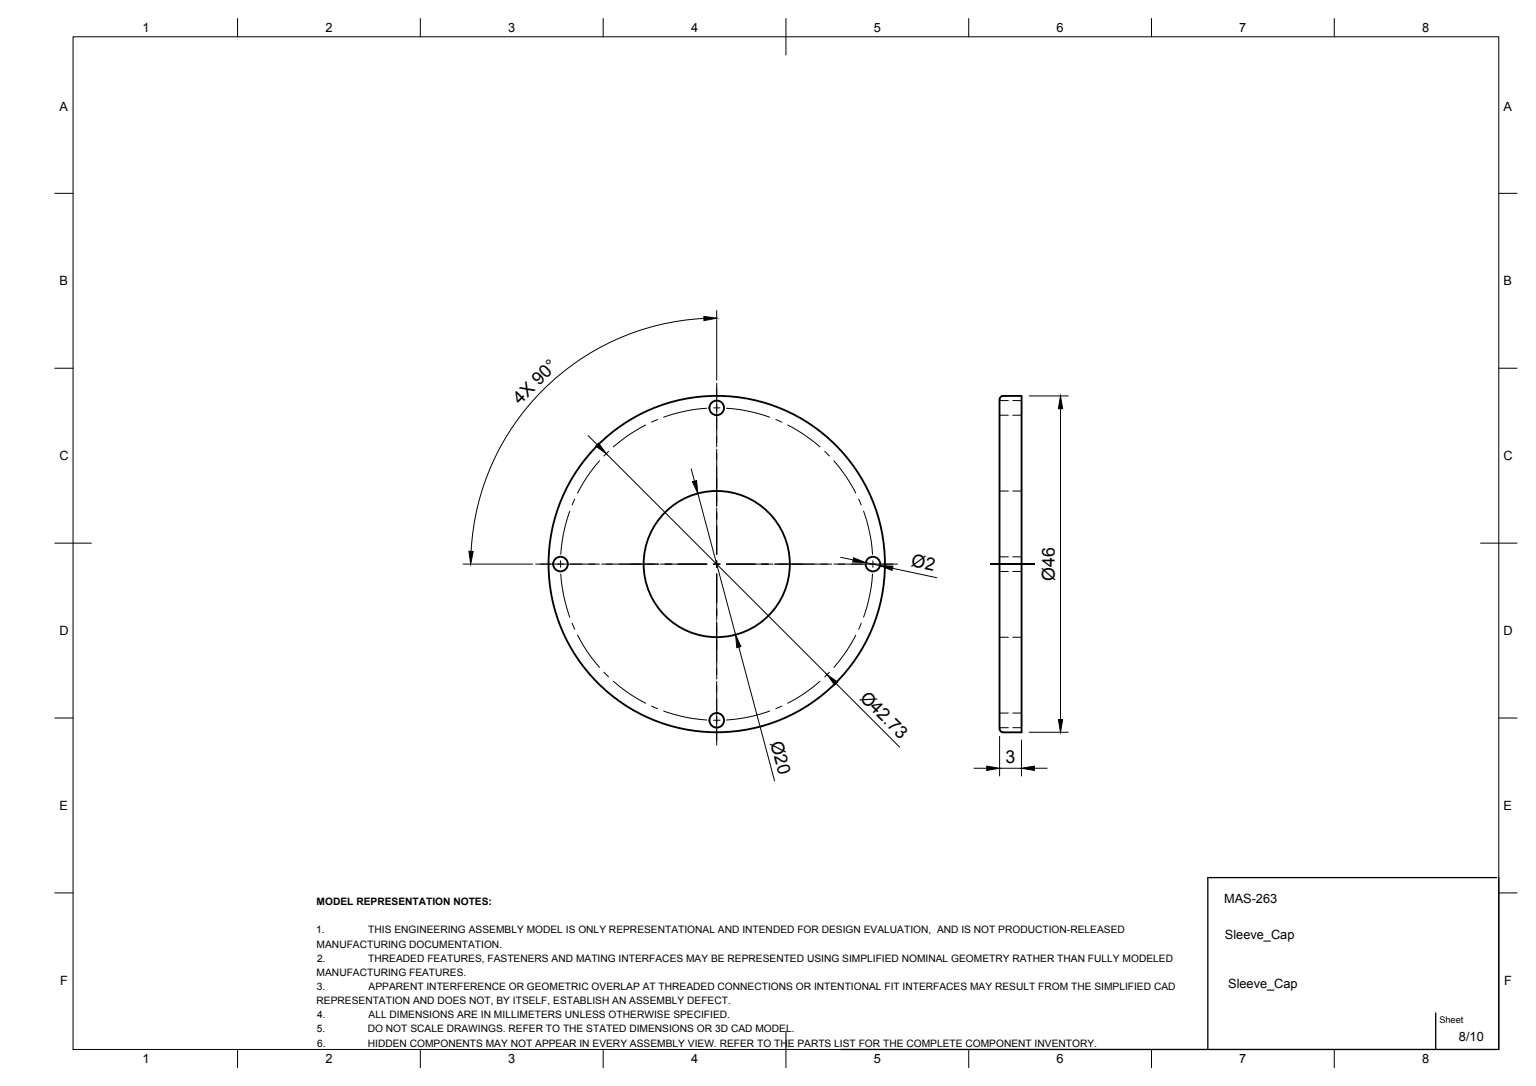
ISO-10303-21;
HEADER;
/* Generated by software containing ST-Developer
 * from STEP Tools, Inc. (www.steptools.com) 
 */

FILE_DESCRIPTION(
/* description */ (''),
/* implementation_level */ '2;1');

FILE_NAME(
/* name */ 'Sleeve_Cap.step',
/* time_stamp */ '2026-10-12T15:47:30-07:00',
/* author */ (''),
/* organization */ (''),
/* preprocessor_version */ 'ST-DEVELOPER v20.2',
/* originating_system */ 'Autodesk Translation Framework v15.15.0.0',
/* authorisation */ '');

FILE_SCHEMA (('AUTOMOTIVE_DESIGN { 1 0 10303 214 3 1 1 }'));
ENDSEC;

DATA;
#10=MECHANICAL_DESIGN_GEOMETRIC_PRESENTATION_REPRESENTATION('',(#86),#88483);
#68=SHAPE_REPRESENTATION_RELATIONSHIP('SRR','None',#88524,#77);
#77=ADVANCED_BREP_SHAPE_REPRESENTATION('',(#121),#88478);
#86=STYLED_ITEM('',(#88574),#121);
#121=MANIFOLD_SOLID_BREP('Body1',#12996);
#173=TOROIDAL_SURFACE('',#13852,22.5,0.5);
#368=FACE_BOUND('',#1937,.T.);
#369=FACE_BOUND('',#1938,.T.);
#370=FACE_BOUND('',#1939,.T.);
#371=FACE_BOUND('',#1940,.T.);
#372=FACE_BOUND('',#1941,.T.);
#373=FACE_BOUND('',#1948,.T.);
#374=FACE_BOUND('',#1949,.T.);
#375=FACE_BOUND('',#1950,.T.);
#376=FACE_BOUND('',#1951,.T.);
#377=FACE_BOUND('',#1952,.T.);
#523=PLANE('',#13859);
#524=PLANE('',#13875);
#1247=FACE_OUTER_BOUND('',#1934,.T.);
#1248=FACE_OUTER_BOUND('',#1935,.T.);
#1249=FACE_OUTER_BOUND('',#1936,.T.);
#1250=FACE_OUTER_BOUND('',#1942,.T.);
#1251=FACE_OUTER_BOUND('',#1943,.T.);
#1252=FACE_OUTER_BOUND('',#1944,.T.);
#1253=FACE_OUTER_BOUND('',#1945,.T.);
#1254=FACE_OUTER_BOUND('',#1946,.T.);
#1255=FACE_OUTER_BOUND('',#1947,.T.);
#1934=EDGE_LOOP('',(#11196,#11197,#11198,#11199,#11200));
#1935=EDGE_LOOP('',(#11201,#11202,#11203,#11204,#11205));
#1936=EDGE_LOOP('',(#11206));
#1937=EDGE_LOOP('',(#11207));
#1938=EDGE_LOOP('',(#11208));
#1939=EDGE_LOOP('',(#11209));
#1940=EDGE_LOOP('',(#11210));
#1941=EDGE_LOOP('',(#11211));
#1942=EDGE_LOOP('',(#11212,#11213,#11214,#11215));
#1943=EDGE_LOOP('',(#11216,#11217,#11218,#11219));
#1944=EDGE_LOOP('',(#11220,#11221,#11222,#11223));
#1945=EDGE_LOOP('',(#11224,#11225,#11226,#11227));
#1946=EDGE_LOOP('',(#11228,#11229,#11230,#11231));
#1947=EDGE_LOOP('',(#11232));
#1948=EDGE_LOOP('',(#11233));
#1949=EDGE_LOOP('',(#11234));
#1950=EDGE_LOOP('',(#11235));
#1951=EDGE_LOOP('',(#11236));
#1952=EDGE_LOOP('',(#11237));
#2625=CIRCLE('',#13853,22.5);
#2626=CIRCLE('',#13854,0.5);
#2627=CIRCLE('',#13855,23.);
#2628=CIRCLE('',#13856,23.);
#2629=CIRCLE('',#13858,23.);
#2630=CIRCLE('',#13860,1.);
#2631=CIRCLE('',#13861,1.);
#2632=CIRCLE('',#13862,1.);
#2633=CIRCLE('',#13863,1.);
#2634=CIRCLE('',#13864,10.);
#2635=CIRCLE('',#13866,1.);
#2636=CIRCLE('',#13868,1.);
#2637=CIRCLE('',#13870,1.);
#2638=CIRCLE('',#13872,1.);
#2639=CIRCLE('',#13874,10.);
#4028=LINE('',#87095,#4498);
#4029=LINE('',#87110,#4499);
#4030=LINE('',#87114,#4500);
#4031=LINE('',#87118,#4501);
#4032=LINE('',#87122,#4502);
#4033=LINE('',#87127,#4503);
#4498=VECTOR('',#16194,23.);
#4499=VECTOR('',#16211,1.);
#4500=VECTOR('',#16216,1.);
#4501=VECTOR('',#16221,1.);
#4502=VECTOR('',#16226,1.);
#4503=VECTOR('',#16233,10.);
#5737=VERTEX_POINT('',#87086);
#5738=VERTEX_POINT('',#87088);
#5739=VERTEX_POINT('',#87090);
#5740=VERTEX_POINT('',#87094);
#5741=VERTEX_POINT('',#87098);
#5742=VERTEX_POINT('',#87100);
#5743=VERTEX_POINT('',#87102);
#5744=VERTEX_POINT('',#87104);
#5745=VERTEX_POINT('',#87106);
#5746=VERTEX_POINT('',#87109);
#5747=VERTEX_POINT('',#87113);
#5748=VERTEX_POINT('',#87117);
#5749=VERTEX_POINT('',#87121);
#5750=VERTEX_POINT('',#87125);
#7610=EDGE_CURVE('',#5737,#5737,#2625,.T.);
#7611=EDGE_CURVE('',#5737,#5738,#2626,.T.);
#7612=EDGE_CURVE('',#5738,#5739,#2627,.T.);
#7613=EDGE_CURVE('',#5739,#5738,#2628,.T.);
#7614=EDGE_CURVE('',#5739,#5740,#4028,.T.);
#7615=EDGE_CURVE('',#5740,#5740,#2629,.T.);
#7616=EDGE_CURVE('',#5741,#5741,#2630,.T.);
#7617=EDGE_CURVE('',#5742,#5742,#2631,.T.);
#7618=EDGE_CURVE('',#5743,#5743,#2632,.T.);
#7619=EDGE_CURVE('',#5744,#5744,#2633,.T.);
#7620=EDGE_CURVE('',#5745,#5745,#2634,.T.);
#7621=EDGE_CURVE('',#5741,#5746,#4029,.T.);
#7622=EDGE_CURVE('',#5746,#5746,#2635,.T.);
#7623=EDGE_CURVE('',#5742,#5747,#4030,.T.);
#7624=EDGE_CURVE('',#5747,#5747,#2636,.T.);
#7625=EDGE_CURVE('',#5743,#5748,#4031,.T.);
#7626=EDGE_CURVE('',#5748,#5748,#2637,.T.);
#7627=EDGE_CURVE('',#5744,#5749,#4032,.T.);
#7628=EDGE_CURVE('',#5749,#5749,#2638,.T.);
#7629=EDGE_CURVE('',#5750,#5750,#2639,.T.);
#7630=EDGE_CURVE('',#5750,#5745,#4033,.T.);
#11196=ORIENTED_EDGE('',*,*,#7610,.T.);
#11197=ORIENTED_EDGE('',*,*,#7611,.T.);
#11198=ORIENTED_EDGE('',*,*,#7612,.T.);
#11199=ORIENTED_EDGE('',*,*,#7613,.T.);
#11200=ORIENTED_EDGE('',*,*,#7611,.F.);
#11201=ORIENTED_EDGE('',*,*,#7613,.F.);
#11202=ORIENTED_EDGE('',*,*,#7614,.T.);
#11203=ORIENTED_EDGE('',*,*,#7615,.T.);
#11204=ORIENTED_EDGE('',*,*,#7614,.F.);
#11205=ORIENTED_EDGE('',*,*,#7612,.F.);
#11206=ORIENTED_EDGE('',*,*,#7610,.F.);
#11207=ORIENTED_EDGE('',*,*,#7616,.T.);
#11208=ORIENTED_EDGE('',*,*,#7617,.T.);
#11209=ORIENTED_EDGE('',*,*,#7618,.T.);
#11210=ORIENTED_EDGE('',*,*,#7619,.T.);
#11211=ORIENTED_EDGE('',*,*,#7620,.T.);
#11212=ORIENTED_EDGE('',*,*,#7616,.F.);
#11213=ORIENTED_EDGE('',*,*,#7621,.T.);
#11214=ORIENTED_EDGE('',*,*,#7622,.F.);
#11215=ORIENTED_EDGE('',*,*,#7621,.F.);
#11216=ORIENTED_EDGE('',*,*,#7617,.F.);
#11217=ORIENTED_EDGE('',*,*,#7623,.T.);
#11218=ORIENTED_EDGE('',*,*,#7624,.F.);
#11219=ORIENTED_EDGE('',*,*,#7623,.F.);
#11220=ORIENTED_EDGE('',*,*,#7618,.F.);
#11221=ORIENTED_EDGE('',*,*,#7625,.T.);
#11222=ORIENTED_EDGE('',*,*,#7626,.F.);
#11223=ORIENTED_EDGE('',*,*,#7625,.F.);
#11224=ORIENTED_EDGE('',*,*,#7619,.F.);
#11225=ORIENTED_EDGE('',*,*,#7627,.T.);
#11226=ORIENTED_EDGE('',*,*,#7628,.F.);
#11227=ORIENTED_EDGE('',*,*,#7627,.F.);
#11228=ORIENTED_EDGE('',*,*,#7629,.T.);
#11229=ORIENTED_EDGE('',*,*,#7630,.T.);
#11230=ORIENTED_EDGE('',*,*,#7620,.F.);
#11231=ORIENTED_EDGE('',*,*,#7630,.F.);
#11232=ORIENTED_EDGE('',*,*,#7615,.F.);
#11233=ORIENTED_EDGE('',*,*,#7629,.F.);
#11234=ORIENTED_EDGE('',*,*,#7628,.T.);
#11235=ORIENTED_EDGE('',*,*,#7626,.T.);
#11236=ORIENTED_EDGE('',*,*,#7624,.T.);
#11237=ORIENTED_EDGE('',*,*,#7622,.T.);
#12245=CYLINDRICAL_SURFACE('',#13857,23.);
#12246=CYLINDRICAL_SURFACE('',#13865,1.);
#12247=CYLINDRICAL_SURFACE('',#13867,1.);
#12248=CYLINDRICAL_SURFACE('',#13869,1.);
#12249=CYLINDRICAL_SURFACE('',#13871,1.);
#12250=CYLINDRICAL_SURFACE('',#13873,10.);
#12777=ADVANCED_FACE('',(#1247),#173,.T.);
#12778=ADVANCED_FACE('',(#1248),#12245,.T.);
#12779=ADVANCED_FACE('',(#1249,#368,#369,#370,#371,#372),#523,.T.);
#12780=ADVANCED_FACE('',(#1250),#12246,.F.);
#12781=ADVANCED_FACE('',(#1251),#12247,.F.);
#12782=ADVANCED_FACE('',(#1252),#12248,.F.);
#12783=ADVANCED_FACE('',(#1253),#12249,.F.);
#12784=ADVANCED_FACE('',(#1254),#12250,.F.);
#12785=ADVANCED_FACE('',(#1255,#373,#374,#375,#376,#377),#524,.F.);
#12996=CLOSED_SHELL('',(#12777,#12778,#12779,#12780,#12781,#12782,#12783,
#12784,#12785));
#13851=AXIS2_PLACEMENT_3D('',#87084,#16180,#16181);
#13852=AXIS2_PLACEMENT_3D('',#87085,#16182,#16183);
#13853=AXIS2_PLACEMENT_3D('',#87087,#16184,#16185);
#13854=AXIS2_PLACEMENT_3D('',#87089,#16186,#16187);
#13855=AXIS2_PLACEMENT_3D('',#87091,#16188,#16189);
#13856=AXIS2_PLACEMENT_3D('',#87092,#16190,#16191);
#13857=AXIS2_PLACEMENT_3D('',#87093,#16192,#16193);
#13858=AXIS2_PLACEMENT_3D('',#87096,#16195,#16196);
#13859=AXIS2_PLACEMENT_3D('',#87097,#16197,#16198);
#13860=AXIS2_PLACEMENT_3D('',#87099,#16199,#16200);
#13861=AXIS2_PLACEMENT_3D('',#87101,#16201,#16202);
#13862=AXIS2_PLACEMENT_3D('',#87103,#16203,#16204);
#13863=AXIS2_PLACEMENT_3D('',#87105,#16205,#16206);
#13864=AXIS2_PLACEMENT_3D('',#87107,#16207,#16208);
#13865=AXIS2_PLACEMENT_3D('',#87108,#16209,#16210);
#13866=AXIS2_PLACEMENT_3D('',#87111,#16212,#16213);
#13867=AXIS2_PLACEMENT_3D('',#87112,#16214,#16215);
#13868=AXIS2_PLACEMENT_3D('',#87115,#16217,#16218);
#13869=AXIS2_PLACEMENT_3D('',#87116,#16219,#16220);
#13870=AXIS2_PLACEMENT_3D('',#87119,#16222,#16223);
#13871=AXIS2_PLACEMENT_3D('',#87120,#16224,#16225);
#13872=AXIS2_PLACEMENT_3D('',#87123,#16227,#16228);
#13873=AXIS2_PLACEMENT_3D('',#87124,#16229,#16230);
#13874=AXIS2_PLACEMENT_3D('',#87126,#16231,#16232);
#13875=AXIS2_PLACEMENT_3D('',#87128,#16234,#16235);
#16180=DIRECTION('axis',(0.,0.,1.));
#16181=DIRECTION('refdir',(1.,0.,0.));
#16182=DIRECTION('center_axis',(0.,0.,1.));
#16183=DIRECTION('ref_axis',(1.,0.,0.));
#16184=DIRECTION('center_axis',(0.,0.,-1.));
#16185=DIRECTION('ref_axis',(-1.,0.,0.));
#16186=DIRECTION('center_axis',(1.22464679914735E-16,-1.,0.));
#16187=DIRECTION('ref_axis',(-1.,-1.22464679914735E-16,0.));
#16188=DIRECTION('center_axis',(0.,0.,1.));
#16189=DIRECTION('ref_axis',(-1.,0.,0.));
#16190=DIRECTION('center_axis',(0.,0.,1.));
#16191=DIRECTION('ref_axis',(-1.,0.,0.));
#16192=DIRECTION('center_axis',(0.,0.,1.));
#16193=DIRECTION('ref_axis',(-1.,0.,0.));
#16194=DIRECTION('',(0.,0.,-1.));
#16195=DIRECTION('center_axis',(0.,0.,1.));
#16196=DIRECTION('ref_axis',(-1.,0.,0.));
#16197=DIRECTION('center_axis',(0.,0.,1.));
#16198=DIRECTION('ref_axis',(-1.,0.,0.));
#16199=DIRECTION('center_axis',(0.,0.,-1.));
#16200=DIRECTION('ref_axis',(-1.,0.,0.));
#16201=DIRECTION('center_axis',(0.,0.,-1.));
#16202=DIRECTION('ref_axis',(-1.,0.,0.));
#16203=DIRECTION('center_axis',(0.,0.,-1.));
#16204=DIRECTION('ref_axis',(-1.,0.,0.));
#16205=DIRECTION('center_axis',(0.,0.,-1.));
#16206=DIRECTION('ref_axis',(-1.,0.,0.));
#16207=DIRECTION('center_axis',(0.,0.,-1.));
#16208=DIRECTION('ref_axis',(-1.,0.,0.));
#16209=DIRECTION('center_axis',(0.,0.,-1.));
#16210=DIRECTION('ref_axis',(-1.,0.,0.));
#16211=DIRECTION('',(0.,0.,-1.));
#16212=DIRECTION('center_axis',(0.,0.,1.));
#16213=DIRECTION('ref_axis',(-1.,0.,0.));
#16214=DIRECTION('center_axis',(0.,0.,-1.));
#16215=DIRECTION('ref_axis',(-1.,0.,0.));
#16216=DIRECTION('',(0.,0.,-1.));
#16217=DIRECTION('center_axis',(0.,0.,1.));
#16218=DIRECTION('ref_axis',(-1.,0.,0.));
#16219=DIRECTION('center_axis',(0.,0.,-1.));
#16220=DIRECTION('ref_axis',(-1.,0.,0.));
#16221=DIRECTION('',(0.,0.,-1.));
#16222=DIRECTION('center_axis',(0.,0.,1.));
#16223=DIRECTION('ref_axis',(-1.,0.,0.));
#16224=DIRECTION('center_axis',(0.,0.,-1.));
#16225=DIRECTION('ref_axis',(-1.,0.,0.));
#16226=DIRECTION('',(0.,0.,-1.));
#16227=DIRECTION('center_axis',(0.,0.,1.));
#16228=DIRECTION('ref_axis',(-1.,0.,0.));
#16229=DIRECTION('center_axis',(0.,0.,1.));
#16230=DIRECTION('ref_axis',(-1.,0.,0.));
#16231=DIRECTION('center_axis',(0.,0.,-1.));
#16232=DIRECTION('ref_axis',(-1.,0.,0.));
#16233=DIRECTION('',(0.,0.,1.));
#16234=DIRECTION('center_axis',(0.,0.,1.));
#16235=DIRECTION('ref_axis',(-1.,0.,0.));
#87084=CARTESIAN_POINT('',(0.,0.,0.));
#87085=CARTESIAN_POINT('Origin',(0.,0.,29.5000004769));
#87086=CARTESIAN_POINT('',(-22.5,-2.75545529808155E-15,30.0000004769));
#87087=CARTESIAN_POINT('Origin',(0.,0.,30.0000004769));
#87088=CARTESIAN_POINT('',(-23.,-2.81668763803891E-15,29.5000004769));
#87089=CARTESIAN_POINT('Origin',(-22.5,-2.75545529808154E-15,29.5000004769));
#87090=CARTESIAN_POINT('',(23.,2.81668763803891E-15,29.5000004769));
#87091=CARTESIAN_POINT('Origin',(0.,0.,29.5000004769));
#87092=CARTESIAN_POINT('Origin',(0.,0.,29.5000004769));
#87093=CARTESIAN_POINT('Origin',(0.,0.,27.0000004769));
#87094=CARTESIAN_POINT('',(23.,2.81668763803891E-15,27.0000004769));
#87095=CARTESIAN_POINT('',(23.,2.81668763803891E-15,27.0000004769));
#87096=CARTESIAN_POINT('Origin',(0.,0.,27.0000004769));
#87097=CARTESIAN_POINT('Origin',(0.,0.,30.0000004769));
#87098=CARTESIAN_POINT('',(-20.3644359551636,4.86632242102517E-15,30.0000004769));
#87099=CARTESIAN_POINT('Origin',(-21.3644359551636,4.74385774111043E-15,
30.0000004769));
#87100=CARTESIAN_POINT('',(1.,21.3644359551636,30.0000004769));
#87101=CARTESIAN_POINT('Origin',(2.61638881080797E-15,21.3644359551636,
30.0000004769));
#87102=CARTESIAN_POINT('',(1.,-21.3644359551636,30.0000004769));
#87103=CARTESIAN_POINT('Origin',(0.,-21.3644359551636,30.0000004769));
#87104=CARTESIAN_POINT('',(22.3644359551636,4.86632242102517E-15,30.0000004769));
#87105=CARTESIAN_POINT('Origin',(21.3644359551636,4.74385774111043E-15,
30.0000004769));
#87106=CARTESIAN_POINT('',(10.,1.22464679914735E-15,30.0000004769));
#87107=CARTESIAN_POINT('Origin',(0.,0.,30.0000004769));
#87108=CARTESIAN_POINT('Origin',(-21.3644359551636,4.74385774111043E-15,
30.0000004769));
#87109=CARTESIAN_POINT('',(-20.3644359551636,4.86632242102517E-15,27.0000004769));
#87110=CARTESIAN_POINT('',(-20.3644359551636,4.62139306119569E-15,30.0000004769));
#87111=CARTESIAN_POINT('Origin',(-21.3644359551636,4.74385774111043E-15,
27.0000004769));
#87112=CARTESIAN_POINT('Origin',(2.61638881080797E-15,21.3644359551636,
30.0000004769));
#87113=CARTESIAN_POINT('',(1.,21.3644359551636,27.0000004769));
#87114=CARTESIAN_POINT('',(1.,21.3644359551636,30.0000004769));
#87115=CARTESIAN_POINT('Origin',(2.61638881080797E-15,21.3644359551636,
27.0000004769));
#87116=CARTESIAN_POINT('Origin',(0.,-21.3644359551636,30.0000004769));
#87117=CARTESIAN_POINT('',(1.,-21.3644359551636,27.0000004769));
#87118=CARTESIAN_POINT('',(1.,-21.3644359551636,30.0000004769));
#87119=CARTESIAN_POINT('Origin',(0.,-21.3644359551636,27.0000004769));
#87120=CARTESIAN_POINT('Origin',(21.3644359551636,4.74385774111043E-15,
30.0000004769));
#87121=CARTESIAN_POINT('',(22.3644359551636,4.86632242102517E-15,27.0000004769));
#87122=CARTESIAN_POINT('',(22.3644359551636,4.62139306119569E-15,30.0000004769));
#87123=CARTESIAN_POINT('Origin',(21.3644359551636,4.74385774111043E-15,
27.0000004769));
#87124=CARTESIAN_POINT('Origin',(0.,0.,27.0000004769));
#87125=CARTESIAN_POINT('',(10.,1.22464679914735E-15,27.0000004769));
#87126=CARTESIAN_POINT('Origin',(0.,0.,27.0000004769));
#87127=CARTESIAN_POINT('',(10.,1.22464679914735E-15,27.0000004769));
#87128=CARTESIAN_POINT('Origin',(0.,0.,27.0000004769));
#88467=UNCERTAINTY_MEASURE_WITH_UNIT(LENGTH_MEASURE(0.01),#88484,
'DISTANCE_ACCURACY_VALUE',
'Maximum model space distance between geometric entities at asserted c
onnectivities');
#88472=UNCERTAINTY_MEASURE_WITH_UNIT(LENGTH_MEASURE(0.01),#88484,
'DISTANCE_ACCURACY_VALUE',
'Maximum model space distance between geometric entities at asserted c
onnectivities');
#88478=(
GEOMETRIC_REPRESENTATION_CONTEXT(3)
GLOBAL_UNCERTAINTY_ASSIGNED_CONTEXT((#88467))
GLOBAL_UNIT_ASSIGNED_CONTEXT((#88484,#88486,#88487))
REPRESENTATION_CONTEXT('','3D')
);
#88483=(
GEOMETRIC_REPRESENTATION_CONTEXT(3)
GLOBAL_UNCERTAINTY_ASSIGNED_CONTEXT((#88472))
GLOBAL_UNIT_ASSIGNED_CONTEXT((#88484,#88486,#88487))
REPRESENTATION_CONTEXT('','3D')
);
#88484=(
LENGTH_UNIT()
NAMED_UNIT(*)
SI_UNIT(.MILLI.,.METRE.)
);
#88486=(
NAMED_UNIT(*)
PLANE_ANGLE_UNIT()
SI_UNIT($,.RADIAN.)
);
#88487=(
NAMED_UNIT(*)
SI_UNIT($,.STERADIAN.)
SOLID_ANGLE_UNIT()
);
#88493=SHAPE_DEFINITION_REPRESENTATION(#88503,#88524);
#88503=PRODUCT_DEFINITION_SHAPE('',$,#88535);
#88524=SHAPE_REPRESENTATION('',(#13851),#88478);
#88529=PRODUCT_DEFINITION_CONTEXT('part definition',#88561,'design');
#88535=PRODUCT_DEFINITION('Sleeve_Cap','Sleeve_Cap',#88545,#88529);
#88545=PRODUCT_DEFINITION_FORMATION('',$,#88568);
#88561=APPLICATION_CONTEXT(
'Core Data for Automotive Mechanical Design Process');
#88562=PRODUCT_CONTEXT('part definition',#88561,'mechanical');
#88568=PRODUCT('Sleeve_Cap','Sleeve_Cap',$,(#88562));
#88574=PRESENTATION_STYLE_ASSIGNMENT((#88576));
#88576=SURFACE_STYLE_USAGE(.BOTH.,#88578);
#88578=SURFACE_SIDE_STYLE('',(#88580));
#88580=SURFACE_STYLE_FILL_AREA(#88582);
#88582=FILL_AREA_STYLE('Opaque(160,160,160)',(#88584));
#88584=FILL_AREA_STYLE_COLOUR('Opaque(160,160,160)',#88586);
#88586=COLOUR_RGB('Opaque(160,160,160)', 0.66274510, 0.83137255, 0.94901961);
ENDSEC;
END-ISO-10303-21;
